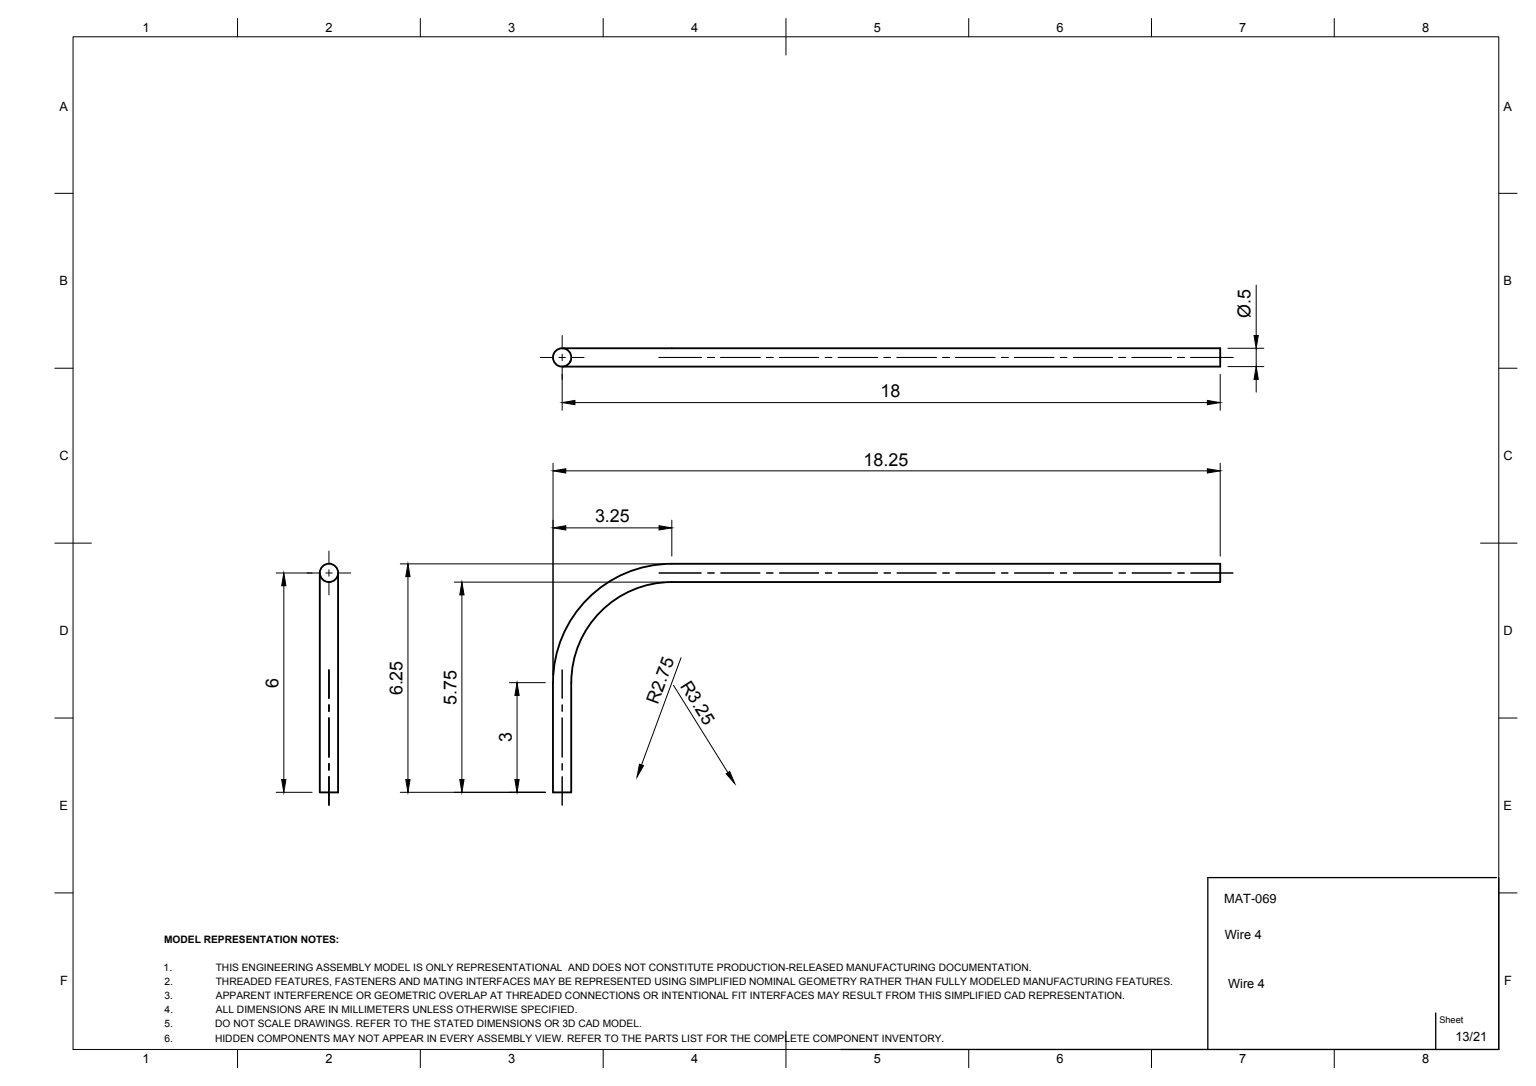
ISO-10303-21;
HEADER;
/* Generated by software containing ST-Developer
 * from STEP Tools, Inc. (www.steptools.com) 
 */

FILE_DESCRIPTION(
/* description */ ('CAx-IF Rec.Pracs.---Representation and Presentation of Product Manufa
cturing Information (PMI)---4.0---2014-10-13'),
/* implementation_level */ '2;1');

FILE_NAME(
/* name */ 'Wire 4.step',
/* time_stamp */ '2026-10-24T15:08:39-07:00',
/* author */ (''),
/* organization */ (''),
/* preprocessor_version */ 'ST-DEVELOPER v20.2',
/* originating_system */ 'Autodesk Translation Framework v15.17.0.0',
/* authorisation */ '');

FILE_SCHEMA (('AP242_MANAGED_MODEL_BASED_3D_ENGINEERING_MIM_LF { 1 0 10303 442 2 1 4 }'));
ENDSEC;

DATA;
#10=MECHANICAL_DESIGN_GEOMETRIC_PRESENTATION_REPRESENTATION('',(#830),#50081);
#776=TOROIDAL_SURFACE('',#10612,0.003,0.00025);
#790=SHAPE_REPRESENTATION_RELATIONSHIP('SRR','None',#50158,#810);
#810=ADVANCED_BREP_SHAPE_REPRESENTATION('',(#850),#50071);
#830=STYLED_ITEM('',(#50260),#850);
#850=MANIFOLD_SOLID_BREP('Body1',#9875);
#997=PLANE('',#10618);
#998=PLANE('',#10619);
#1386=FACE_OUTER_BOUND('',#1965,.T.);
#1387=FACE_OUTER_BOUND('',#1966,.T.);
#1388=FACE_OUTER_BOUND('',#1967,.T.);
#1389=FACE_OUTER_BOUND('',#1968,.T.);
#1390=FACE_OUTER_BOUND('',#1969,.T.);
#1965=EDGE_LOOP('',(#7740,#7741,#7742,#7743,#7744));
#1966=EDGE_LOOP('',(#7745,#7746,#7747,#7748,#7749,#7750));
#1967=EDGE_LOOP('',(#7751,#7752,#7753,#7754,#7755));
#1968=EDGE_LOOP('',(#7756));
#1969=EDGE_LOOP('',(#7757));
#2521=LINE('',#34770,#3099);
#2522=LINE('',#34782,#3100);
#3099=VECTOR('',#12321,0.00025);
#3100=VECTOR('',#12336,0.00025);
#3594=CIRCLE('',#10609,0.00025000000001);
#3595=CIRCLE('',#10610,0.00025000000001);
#3596=CIRCLE('',#10611,0.00025000000001);
#3597=CIRCLE('',#10613,0.00275);
#3598=CIRCLE('',#10614,0.00025000000001);
#3599=CIRCLE('',#10615,0.00025000000001);
#3600=CIRCLE('',#10617,0.00025000000001);
#4289=VERTEX_POINT('',#34767);
#4290=VERTEX_POINT('',#34769);
#4291=VERTEX_POINT('',#34771);
#4292=VERTEX_POINT('',#34775);
#4293=VERTEX_POINT('',#34777);
#4294=VERTEX_POINT('',#34781);
#5523=EDGE_CURVE('',#4289,#4289,#3594,.T.);
#5524=EDGE_CURVE('',#4289,#4290,#2521,.T.);
#5525=EDGE_CURVE('',#4290,#4291,#3595,.T.);
#5526=EDGE_CURVE('',#4291,#4290,#3596,.T.);
#5527=EDGE_CURVE('',#4291,#4292,#3597,.T.);
#5528=EDGE_CURVE('',#4292,#4293,#3598,.T.);
#5529=EDGE_CURVE('',#4293,#4292,#3599,.T.);
#5530=EDGE_CURVE('',#4293,#4294,#2522,.T.);
#5531=EDGE_CURVE('',#4294,#4294,#3600,.T.);
#7740=ORIENTED_EDGE('',*,*,#5523,.F.);
#7741=ORIENTED_EDGE('',*,*,#5524,.T.);
#7742=ORIENTED_EDGE('',*,*,#5525,.T.);
#7743=ORIENTED_EDGE('',*,*,#5526,.T.);
#7744=ORIENTED_EDGE('',*,*,#5524,.F.);
#7745=ORIENTED_EDGE('',*,*,#5526,.F.);
#7746=ORIENTED_EDGE('',*,*,#5527,.T.);
#7747=ORIENTED_EDGE('',*,*,#5528,.T.);
#7748=ORIENTED_EDGE('',*,*,#5529,.T.);
#7749=ORIENTED_EDGE('',*,*,#5527,.F.);
#7750=ORIENTED_EDGE('',*,*,#5525,.F.);
#7751=ORIENTED_EDGE('',*,*,#5529,.F.);
#7752=ORIENTED_EDGE('',*,*,#5530,.T.);
#7753=ORIENTED_EDGE('',*,*,#5531,.T.);
#7754=ORIENTED_EDGE('',*,*,#5530,.F.);
#7755=ORIENTED_EDGE('',*,*,#5528,.F.);
#7756=ORIENTED_EDGE('',*,*,#5523,.T.);
#7757=ORIENTED_EDGE('',*,*,#5531,.F.);
#9240=CYLINDRICAL_SURFACE('',#10608,0.00025);
#9241=CYLINDRICAL_SURFACE('',#10616,0.00025);
#9608=ADVANCED_FACE('',(#1386),#9240,.T.);
#9609=ADVANCED_FACE('',(#1387),#776,.T.);
#9610=ADVANCED_FACE('',(#1388),#9241,.T.);
#9611=ADVANCED_FACE('',(#1389),#997,.T.);
#9612=ADVANCED_FACE('',(#1390),#998,.F.);
#9875=CLOSED_SHELL('',(#9608,#9609,#9610,#9611,#9612));
#10607=AXIS2_PLACEMENT_3D('',#34765,#12315,#12316);
#10608=AXIS2_PLACEMENT_3D('',#34766,#12317,#12318);
#10609=AXIS2_PLACEMENT_3D('',#34768,#12319,#12320);
#10610=AXIS2_PLACEMENT_3D('',#34772,#12322,#12323);
#10611=AXIS2_PLACEMENT_3D('',#34773,#12324,#12325);
#10612=AXIS2_PLACEMENT_3D('',#34774,#12326,#12327);
#10613=AXIS2_PLACEMENT_3D('',#34776,#12328,#12329);
#10614=AXIS2_PLACEMENT_3D('',#34778,#12330,#12331);
#10615=AXIS2_PLACEMENT_3D('',#34779,#12332,#12333);
#10616=AXIS2_PLACEMENT_3D('',#34780,#12334,#12335);
#10617=AXIS2_PLACEMENT_3D('',#34783,#12337,#12338);
#10618=AXIS2_PLACEMENT_3D('',#34784,#12339,#12340);
#10619=AXIS2_PLACEMENT_3D('',#34785,#12341,#12342);
#12315=DIRECTION('axis',(0.,0.,1.));
#12316=DIRECTION('refdir',(1.,0.,0.));
#12317=DIRECTION('center_axis',(2.42833204006769E-16,2.41473507855972E-15,
-1.));
#12318=DIRECTION('ref_axis',(0.422618261740706,0.906307787036647,2.29111895189949E-15));
#12319=DIRECTION('center_axis',(3.62526098085663E-11,-1.69023416117786E-11,
-1.));
#12320=DIRECTION('ref_axis',(0.422618261740706,0.906307787036647,2.29111895186089E-15));
#12321=DIRECTION('',(-2.42833204006769E-16,-2.41473507855972E-15,1.));
#12322=DIRECTION('center_axis',(3.62526098085663E-11,-1.69023416117786E-11,
-1.));
#12323=DIRECTION('ref_axis',(0.422618261740706,0.906307787036647,2.29111895186089E-15));
#12324=DIRECTION('center_axis',(3.62526098085663E-11,-1.69023416117786E-11,
-1.));
#12325=DIRECTION('ref_axis',(0.422618261740706,0.906307787036647,2.29111895186089E-15));
#12326=DIRECTION('center_axis',(0.422618261740706,0.906307787036647,1.97116866169388E-15));
#12327=DIRECTION('ref_axis',(1.33440267382831E-16,2.1350442781253E-15,-1.));
#12328=DIRECTION('center_axis',(-0.422618261740706,-0.906307787036647,-1.97116866169388E-15));
#12329=DIRECTION('ref_axis',(3.8032634610719E-16,1.99759488807599E-15,-1.));
#12330=DIRECTION('center_axis',(0.906307787036647,-0.422618261740706,-8.00429517722823E-16));
#12331=DIRECTION('ref_axis',(0.422618261740706,0.906307787036647,1.97116866169388E-15));
#12332=DIRECTION('center_axis',(0.906307787036647,-0.422618261740706,-8.00429517722823E-16));
#12333=DIRECTION('ref_axis',(0.422618261740706,0.906307787036647,1.97116866169388E-15));
#12334=DIRECTION('center_axis',(0.906307787036647,-0.422618261740706,-8.00429517722823E-16));
#12335=DIRECTION('ref_axis',(0.422618261740706,0.906307787036647,1.97116866169388E-15));
#12336=DIRECTION('',(-0.906307787036647,0.422618261740706,8.00429517722823E-16));
#12337=DIRECTION('center_axis',(0.906307787036647,-0.422618261740706,-8.00429517722823E-16));
#12338=DIRECTION('ref_axis',(0.422618261740706,0.906307787036647,1.97116866169388E-15));
#12339=DIRECTION('center_axis',(2.98328550528607E-16,2.38885717348462E-15,
-1.));
#12340=DIRECTION('ref_axis',(0.906307787036647,-0.422618261740706,-7.39197177765454E-16));
#12341=DIRECTION('center_axis',(0.906307787036647,-0.422618261740706,-8.00429517722823E-16));
#12342=DIRECTION('ref_axis',(2.42833204006769E-16,2.41473507855972E-15,
-1.));
#34765=CARTESIAN_POINT('',(0.,0.,0.));
#34766=CARTESIAN_POINT('Origin',(0.00578869086912964,-0.0359819282833906,
-0.0013758532865581));
#34767=CARTESIAN_POINT('',(0.00568303630369446,-0.0362085052301498,-0.0043758532865581));
#34768=CARTESIAN_POINT('Origin',(0.00578869086912542,-0.0359819282833998,
-0.0043758532865481));
#34769=CARTESIAN_POINT('',(0.00568303630369446,-0.0362085052301498,-0.0013758532865381));
#34770=CARTESIAN_POINT('',(0.00568303630369446,-0.0362085052301498,-0.0013758532865581));
#34771=CARTESIAN_POINT('',(0.00556211392236143,-0.0358762737179513,-0.0013758532865581));
#34772=CARTESIAN_POINT('Origin',(0.00578869086912542,-0.0359819282833998,
-0.0013758532865481));
#34773=CARTESIAN_POINT('Origin',(0.00578869086912542,-0.0359819282833998,
-0.0013758532865481));
#34774=CARTESIAN_POINT('Origin',(0.0030697675080197,-0.0347140734981686,
-0.0013758532865581));
#34775=CARTESIAN_POINT('',(0.00306976750801062,-0.0347140734981644,0.0013741467134419));
#34776=CARTESIAN_POINT('Origin',(0.0030697675080197,-0.0347140734981686,
-0.0013758532865581));
#34777=CARTESIAN_POINT('',(0.0029641129425755,-0.0349406504449234,0.0016241467134419));
#34778=CARTESIAN_POINT('Origin',(0.00306976750800641,-0.0347140734981734,
0.0016241467134519));
#34779=CARTESIAN_POINT('Origin',(0.00306976750800641,-0.0347140734981734,
0.0016241467134519));
#34780=CARTESIAN_POINT('Origin',(-0.01052484929753,-0.0283747995720579,
0.00162414671344191));
#34781=CARTESIAN_POINT('',(-0.0106305038629742,-0.0286013765188128,0.00162414671344191));
#34782=CARTESIAN_POINT('',(-0.0106305038629652,-0.0286013765188171,0.00162414671344191));
#34783=CARTESIAN_POINT('Origin',(-0.0105248492975433,-0.0283747995720628,
0.00162414671345191));
#34784=CARTESIAN_POINT('Origin',(0.00578869086912964,-0.0359819282833906,
-0.0043758532865581));
#34785=CARTESIAN_POINT('Origin',(-0.01052484929753,-0.0283747995720579,
0.00162414671344191));
#50049=UNCERTAINTY_MEASURE_WITH_UNIT(LENGTH_MEASURE(1.E-5),#50082,
'DISTANCE_ACCURACY_VALUE',
'Maximum model space distance between geometric entities at asserted c
onnectivities');
#50059=UNCERTAINTY_MEASURE_WITH_UNIT(LENGTH_MEASURE(1.E-5),#50082,
'DISTANCE_ACCURACY_VALUE',
'Maximum model space distance between geometric entities at asserted c
onnectivities');
#50071=(
GEOMETRIC_REPRESENTATION_CONTEXT(3)
GLOBAL_UNCERTAINTY_ASSIGNED_CONTEXT((#50049))
GLOBAL_UNIT_ASSIGNED_CONTEXT((#50082,#50083,#50084))
REPRESENTATION_CONTEXT('','3D')
);
#50081=(
GEOMETRIC_REPRESENTATION_CONTEXT(3)
GLOBAL_UNCERTAINTY_ASSIGNED_CONTEXT((#50059))
GLOBAL_UNIT_ASSIGNED_CONTEXT((#50082,#50083,#50084))
REPRESENTATION_CONTEXT('','3D')
);
#50082=(
LENGTH_UNIT()
NAMED_UNIT(*)
SI_UNIT($,.METRE.)
);
#50083=(
NAMED_UNIT(*)
PLANE_ANGLE_UNIT()
SI_UNIT($,.RADIAN.)
);
#50084=(
NAMED_UNIT(*)
SI_UNIT($,.STERADIAN.)
SOLID_ANGLE_UNIT()
);
#50096=SHAPE_DEFINITION_REPRESENTATION(#50117,#50158);
#50117=PRODUCT_DEFINITION_SHAPE('',$,#50180);
#50158=SHAPE_REPRESENTATION('',(#10607),#50071);
#50168=PRODUCT_DEFINITION_CONTEXT('part definition',#50233,'design');
#50180=PRODUCT_DEFINITION('Wire 4','Wire 4',#50201,#50168);
#50201=PRODUCT_DEFINITION_FORMATION('',$,#50246);
#50233=APPLICATION_CONTEXT('Managed model based 3d engineering');
#50234=PRODUCT_CONTEXT('part definition',#50233,'mechanical');
#50246=PRODUCT('Wire 4','Wire 4',
'LEGAL AND USAGE DISCLAIMER: this Data/Model is provided \X2\201C\X0\A
S IS\X2\201D\X0\ for informational and representational only. It is a 
geometric approximation and is NOT engineered, certified, or guarantee
d for dimensional accuracy, exact tolerances, or production-level prec
ision. Vendor disclaims all implied warranties including fitness for a
 particular purpose. DO NOT USE FOR DIRECT PHYSICAL MANUFACTURING, AUT
OMATED PRODUCTION, OR SAFETY-CRITICAL SYSTEMS without independent engi
neering verification and resolution of any design discrepancies.',(#50234));
#50260=PRESENTATION_STYLE_ASSIGNMENT((#50267));
#50267=SURFACE_STYLE_USAGE(.BOTH.,#50274);
#50274=SURFACE_SIDE_STYLE('',(#50281));
#50281=SURFACE_STYLE_FILL_AREA(#50288);
#50288=FILL_AREA_STYLE('Opaque(25,25,25)',(#50295));
#50295=FILL_AREA_STYLE_COLOUR('Opaque(25,25,25)',#50302);
#50302=COLOUR_RGB('Opaque(25,25,25)',0.0980392156862745,0.0980392156862745,
0.0980392156862745);
ENDSEC;
END-ISO-10303-21;
